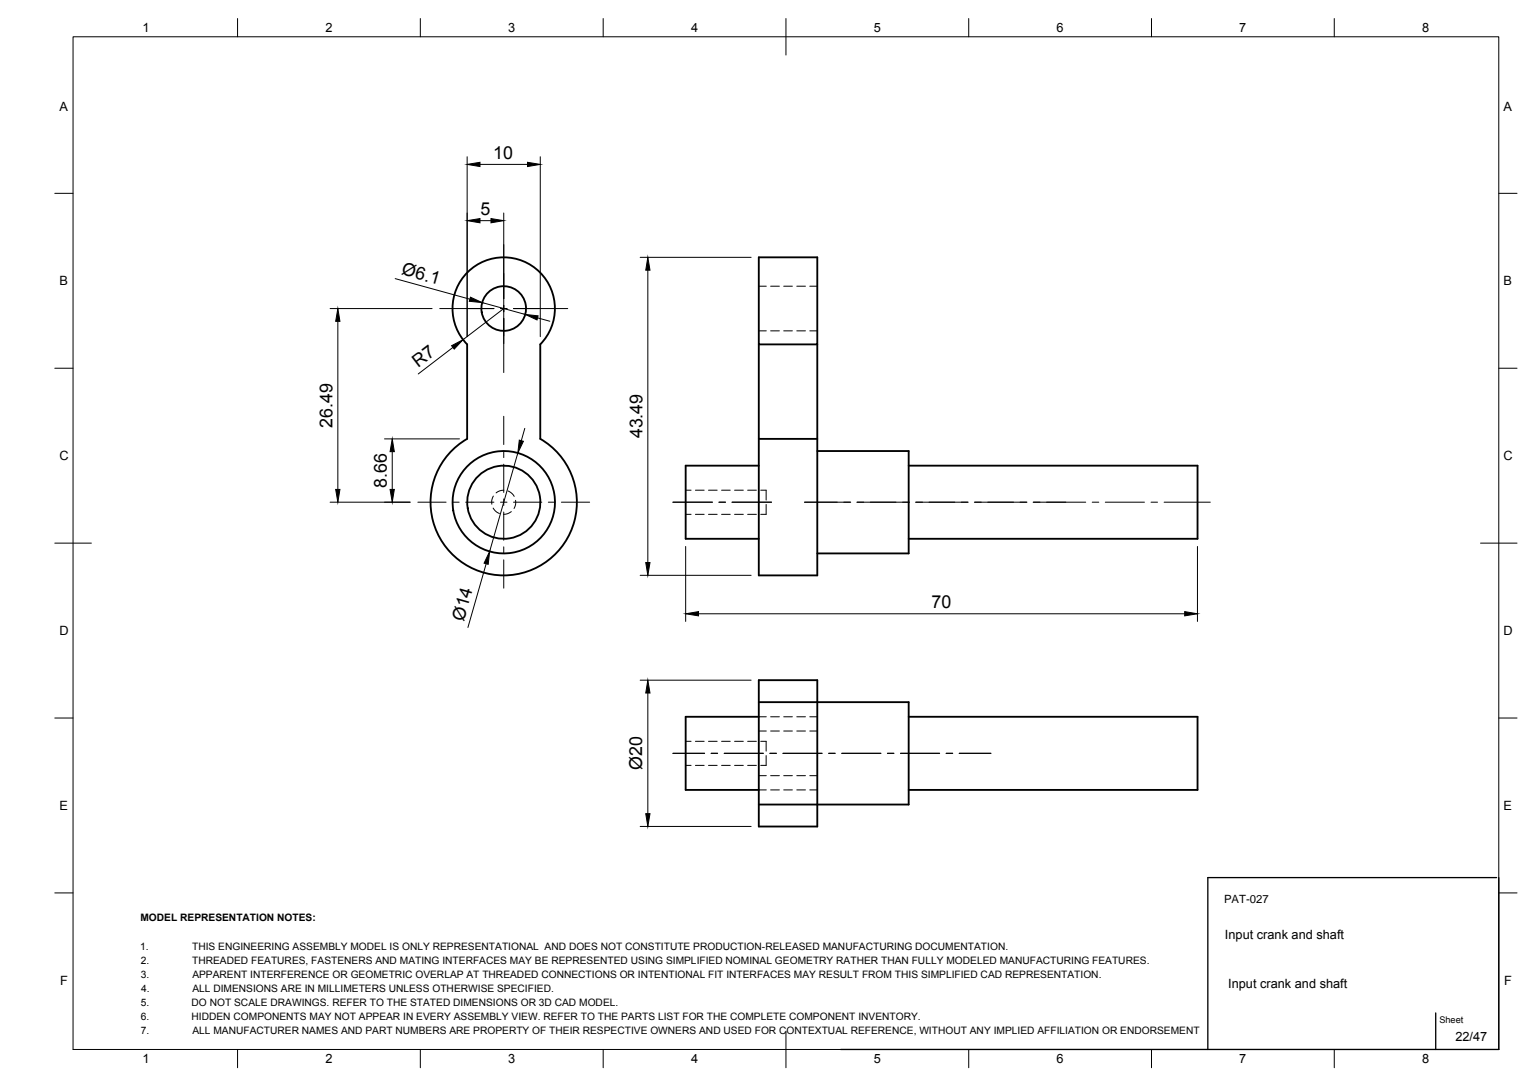
ISO-10303-21;
HEADER;
/* Generated by software containing ST-Developer
 * from STEP Tools, Inc. (www.steptools.com) 
 */

FILE_DESCRIPTION(
/* description */ ('Crank-driven oscillating fan base (mechanism only)'),

/* implementation_level */ '2;1');

FILE_NAME(
/* name */ 'Input crank and shaft.step',
/* time_stamp */ '2026-10-28T03:25:00-07:00',
/* author */ (''),
/* organization */ (''),
/* preprocessor_version */ 'ST-DEVELOPER v20.2',
/* originating_system */ 'Autodesk Translation Framework v15.17.0.0',
/* authorisation */ '');

FILE_SCHEMA (('AUTOMOTIVE_DESIGN { 1 0 10303 214 3 1 1 }'));
ENDSEC;

DATA;
#10=MECHANICAL_DESIGN_GEOMETRIC_PRESENTATION_REPRESENTATION('',(#459),#11916);
#371=SHAPE_REPRESENTATION_RELATIONSHIP('SRR','None',#12097,#411);
#411=ADVANCED_BREP_SHAPE_REPRESENTATION('',(#506),#11888);
#459=STYLED_ITEM('',(#12375),#506);
#506=MANIFOLD_SOLID_BREP('Body1',#6090);
#616=FACE_BOUND('',#1528,.T.);
#617=FACE_BOUND('',#1529,.T.);
#618=FACE_BOUND('',#1533,.T.);
#619=FACE_BOUND('',#1534,.T.);
#620=FACE_BOUND('',#1536,.T.);
#621=FACE_BOUND('',#1541,.T.);
#770=PLANE('',#6968);
#771=PLANE('',#6975);
#772=PLANE('',#6976);
#773=PLANE('',#6979);
#774=PLANE('',#6982);
#775=PLANE('',#6984);
#776=PLANE('',#6992);
#777=PLANE('',#6993);
#1061=FACE_OUTER_BOUND('',#1522,.T.);
#1062=FACE_OUTER_BOUND('',#1523,.T.);
#1063=FACE_OUTER_BOUND('',#1524,.T.);
#1064=FACE_OUTER_BOUND('',#1525,.T.);
#1065=FACE_OUTER_BOUND('',#1526,.T.);
#1066=FACE_OUTER_BOUND('',#1527,.T.);
#1067=FACE_OUTER_BOUND('',#1530,.T.);
#1068=FACE_OUTER_BOUND('',#1531,.T.);
#1069=FACE_OUTER_BOUND('',#1532,.T.);
#1070=FACE_OUTER_BOUND('',#1535,.T.);
#1071=FACE_OUTER_BOUND('',#1537,.T.);
#1072=FACE_OUTER_BOUND('',#1538,.T.);
#1073=FACE_OUTER_BOUND('',#1539,.T.);
#1074=FACE_OUTER_BOUND('',#1540,.T.);
#1075=FACE_OUTER_BOUND('',#1542,.T.);
#1522=EDGE_LOOP('',(#4816,#4817,#4818,#4819));
#1523=EDGE_LOOP('',(#4820));
#1524=EDGE_LOOP('',(#4821,#4822,#4823,#4824));
#1525=EDGE_LOOP('',(#4825,#4826,#4827,#4828));
#1526=EDGE_LOOP('',(#4829,#4830,#4831,#4832));
#1527=EDGE_LOOP('',(#4833,#4834,#4835,#4836));
#1528=EDGE_LOOP('',(#4837));
#1529=EDGE_LOOP('',(#4838));
#1530=EDGE_LOOP('',(#4839,#4840,#4841,#4842));
#1531=EDGE_LOOP('',(#4843,#4844,#4845,#4846));
#1532=EDGE_LOOP('',(#4847,#4848,#4849,#4850));
#1533=EDGE_LOOP('',(#4851));
#1534=EDGE_LOOP('',(#4852));
#1535=EDGE_LOOP('',(#4853));
#1536=EDGE_LOOP('',(#4854));
#1537=EDGE_LOOP('',(#4855,#4856,#4857,#4858));
#1538=EDGE_LOOP('',(#4859,#4860,#4861,#4862));
#1539=EDGE_LOOP('',(#4863,#4864,#4865,#4866));
#1540=EDGE_LOOP('',(#4867));
#1541=EDGE_LOOP('',(#4868));
#1542=EDGE_LOOP('',(#4869));
#1939=LINE('',#10758,#2272);
#1940=LINE('',#10765,#2273);
#1941=LINE('',#10770,#2274);
#1942=LINE('',#10774,#2275);
#1943=LINE('',#10778,#2276);
#1944=LINE('',#10780,#2277);
#1945=LINE('',#10781,#2278);
#1946=LINE('',#10784,#2279);
#1947=LINE('',#10790,#2280);
#1948=LINE('',#10791,#2281);
#1949=LINE('',#10803,#2282);
#1950=LINE('',#10806,#2283);
#1951=LINE('',#10811,#2284);
#2272=VECTOR('',#8368,0.165);
#2273=VECTOR('',#8377,0.305);
#2274=VECTOR('',#8382,1.);
#2275=VECTOR('',#8385,1.);
#2276=VECTOR('',#8390,1.);
#2277=VECTOR('',#8391,1.);
#2278=VECTOR('',#8392,1.);
#2279=VECTOR('',#8395,1.);
#2280=VECTOR('',#8402,1.);
#2281=VECTOR('',#8403,1.);
#2282=VECTOR('',#8420,0.7);
#2283=VECTOR('',#8423,0.5);
#2284=VECTOR('',#8430,0.5);
#2671=CIRCLE('',#6966,0.165);
#2672=CIRCLE('',#6967,0.165);
#2673=CIRCLE('',#6970,0.305);
#2674=CIRCLE('',#6971,0.305);
#2675=CIRCLE('',#6973,0.7);
#2676=CIRCLE('',#6974,0.7);
#2677=CIRCLE('',#6977,1.);
#2678=CIRCLE('',#6978,0.5);
#2679=CIRCLE('',#6981,1.);
#2680=CIRCLE('',#6983,0.7);
#2681=CIRCLE('',#6985,0.7);
#2682=CIRCLE('',#6986,0.5);
#2683=CIRCLE('',#6989,0.5);
#2684=CIRCLE('',#6991,0.5);
#3088=VERTEX_POINT('',#10755);
#3089=VERTEX_POINT('',#10757);
#3090=VERTEX_POINT('',#10762);
#3091=VERTEX_POINT('',#10764);
#3092=VERTEX_POINT('',#10768);
#3093=VERTEX_POINT('',#10769);
#3094=VERTEX_POINT('',#10771);
#3095=VERTEX_POINT('',#10773);
#3096=VERTEX_POINT('',#10777);
#3097=VERTEX_POINT('',#10779);
#3098=VERTEX_POINT('',#10783);
#3099=VERTEX_POINT('',#10786);
#3100=VERTEX_POINT('',#10789);
#3101=VERTEX_POINT('',#10795);
#3102=VERTEX_POINT('',#10798);
#3103=VERTEX_POINT('',#10800);
#3104=VERTEX_POINT('',#10805);
#3105=VERTEX_POINT('',#10809);
#3703=EDGE_CURVE('',#3088,#3088,#2671,.T.);
#3704=EDGE_CURVE('',#3088,#3089,#1939,.T.);
#3705=EDGE_CURVE('',#3089,#3089,#2672,.T.);
#3706=EDGE_CURVE('',#3090,#3090,#2673,.T.);
#3707=EDGE_CURVE('',#3090,#3091,#1940,.T.);
#3708=EDGE_CURVE('',#3091,#3091,#2674,.T.);
#3709=EDGE_CURVE('',#3092,#3093,#1941,.T.);
#3710=EDGE_CURVE('',#3092,#3094,#2675,.T.);
#3711=EDGE_CURVE('',#3095,#3094,#1942,.T.);
#3712=EDGE_CURVE('',#3093,#3095,#2676,.T.);
#3713=EDGE_CURVE('',#3096,#3093,#1943,.T.);
#3714=EDGE_CURVE('',#3097,#3096,#1944,.T.);
#3715=EDGE_CURVE('',#3092,#3097,#1945,.T.);
#3716=EDGE_CURVE('',#3095,#3098,#1946,.T.);
#3717=EDGE_CURVE('',#3098,#3096,#2677,.T.);
#3718=EDGE_CURVE('',#3099,#3099,#2678,.T.);
#3719=EDGE_CURVE('',#3100,#3094,#1947,.T.);
#3720=EDGE_CURVE('',#3098,#3100,#1948,.T.);
#3721=EDGE_CURVE('',#3100,#3097,#2679,.T.);
#3722=EDGE_CURVE('',#3101,#3101,#2680,.T.);
#3723=EDGE_CURVE('',#3102,#3102,#2681,.T.);
#3724=EDGE_CURVE('',#3103,#3103,#2682,.T.);
#3725=EDGE_CURVE('',#3101,#3102,#1949,.T.);
#3726=EDGE_CURVE('',#3103,#3104,#1950,.T.);
#3727=EDGE_CURVE('',#3104,#3104,#2683,.T.);
#3728=EDGE_CURVE('',#3105,#3105,#2684,.T.);
#3729=EDGE_CURVE('',#3105,#3099,#1951,.T.);
#4816=ORIENTED_EDGE('',*,*,#3703,.F.);
#4817=ORIENTED_EDGE('',*,*,#3704,.T.);
#4818=ORIENTED_EDGE('',*,*,#3705,.F.);
#4819=ORIENTED_EDGE('',*,*,#3704,.F.);
#4820=ORIENTED_EDGE('',*,*,#3703,.T.);
#4821=ORIENTED_EDGE('',*,*,#3706,.F.);
#4822=ORIENTED_EDGE('',*,*,#3707,.T.);
#4823=ORIENTED_EDGE('',*,*,#3708,.F.);
#4824=ORIENTED_EDGE('',*,*,#3707,.F.);
#4825=ORIENTED_EDGE('',*,*,#3709,.F.);
#4826=ORIENTED_EDGE('',*,*,#3710,.T.);
#4827=ORIENTED_EDGE('',*,*,#3711,.F.);
#4828=ORIENTED_EDGE('',*,*,#3712,.F.);
#4829=ORIENTED_EDGE('',*,*,#3709,.T.);
#4830=ORIENTED_EDGE('',*,*,#3713,.F.);
#4831=ORIENTED_EDGE('',*,*,#3714,.F.);
#4832=ORIENTED_EDGE('',*,*,#3715,.F.);
#4833=ORIENTED_EDGE('',*,*,#3712,.T.);
#4834=ORIENTED_EDGE('',*,*,#3716,.T.);
#4835=ORIENTED_EDGE('',*,*,#3717,.T.);
#4836=ORIENTED_EDGE('',*,*,#3713,.T.);
#4837=ORIENTED_EDGE('',*,*,#3708,.T.);
#4838=ORIENTED_EDGE('',*,*,#3718,.F.);
#4839=ORIENTED_EDGE('',*,*,#3711,.T.);
#4840=ORIENTED_EDGE('',*,*,#3719,.F.);
#4841=ORIENTED_EDGE('',*,*,#3720,.F.);
#4842=ORIENTED_EDGE('',*,*,#3716,.F.);
#4843=ORIENTED_EDGE('',*,*,#3720,.T.);
#4844=ORIENTED_EDGE('',*,*,#3721,.T.);
#4845=ORIENTED_EDGE('',*,*,#3714,.T.);
#4846=ORIENTED_EDGE('',*,*,#3717,.F.);
#4847=ORIENTED_EDGE('',*,*,#3715,.T.);
#4848=ORIENTED_EDGE('',*,*,#3721,.F.);
#4849=ORIENTED_EDGE('',*,*,#3719,.T.);
#4850=ORIENTED_EDGE('',*,*,#3710,.F.);
#4851=ORIENTED_EDGE('',*,*,#3706,.T.);
#4852=ORIENTED_EDGE('',*,*,#3722,.T.);
#4853=ORIENTED_EDGE('',*,*,#3723,.F.);
#4854=ORIENTED_EDGE('',*,*,#3724,.F.);
#4855=ORIENTED_EDGE('',*,*,#3722,.F.);
#4856=ORIENTED_EDGE('',*,*,#3725,.T.);
#4857=ORIENTED_EDGE('',*,*,#3723,.T.);
#4858=ORIENTED_EDGE('',*,*,#3725,.F.);
#4859=ORIENTED_EDGE('',*,*,#3724,.T.);
#4860=ORIENTED_EDGE('',*,*,#3726,.T.);
#4861=ORIENTED_EDGE('',*,*,#3727,.T.);
#4862=ORIENTED_EDGE('',*,*,#3726,.F.);
#4863=ORIENTED_EDGE('',*,*,#3728,.F.);
#4864=ORIENTED_EDGE('',*,*,#3729,.T.);
#4865=ORIENTED_EDGE('',*,*,#3718,.T.);
#4866=ORIENTED_EDGE('',*,*,#3729,.F.);
#4867=ORIENTED_EDGE('',*,*,#3728,.T.);
#4868=ORIENTED_EDGE('',*,*,#3705,.T.);
#4869=ORIENTED_EDGE('',*,*,#3727,.F.);
#5618=CYLINDRICAL_SURFACE('',#6965,0.165);
#5619=CYLINDRICAL_SURFACE('',#6969,0.305);
#5620=CYLINDRICAL_SURFACE('',#6972,0.7);
#5621=CYLINDRICAL_SURFACE('',#6980,1.);
#5622=CYLINDRICAL_SURFACE('',#6987,0.7);
#5623=CYLINDRICAL_SURFACE('',#6988,0.5);
#5624=CYLINDRICAL_SURFACE('',#6990,0.5);
#5867=ADVANCED_FACE('',(#1061),#5618,.F.);
#5868=ADVANCED_FACE('',(#1062),#770,.T.);
#5869=ADVANCED_FACE('',(#1063),#5619,.F.);
#5870=ADVANCED_FACE('',(#1064),#5620,.T.);
#5871=ADVANCED_FACE('',(#1065),#771,.T.);
#5872=ADVANCED_FACE('',(#1066,#616,#617),#772,.T.);
#5873=ADVANCED_FACE('',(#1067),#773,.T.);
#5874=ADVANCED_FACE('',(#1068),#5621,.T.);
#5875=ADVANCED_FACE('',(#1069,#618,#619),#774,.F.);
#5876=ADVANCED_FACE('',(#1070,#620),#775,.F.);
#5877=ADVANCED_FACE('',(#1071),#5622,.T.);
#5878=ADVANCED_FACE('',(#1072),#5623,.T.);
#5879=ADVANCED_FACE('',(#1073),#5624,.T.);
#5880=ADVANCED_FACE('',(#1074,#621),#776,.T.);
#5881=ADVANCED_FACE('',(#1075),#777,.F.);
#6090=CLOSED_SHELL('',(#5867,#5868,#5869,#5870,#5871,#5872,#5873,#5874,
#5875,#5876,#5877,#5878,#5879,#5880,#5881));
#6964=AXIS2_PLACEMENT_3D('',#10753,#8362,#8363);
#6965=AXIS2_PLACEMENT_3D('',#10754,#8364,#8365);
#6966=AXIS2_PLACEMENT_3D('',#10756,#8366,#8367);
#6967=AXIS2_PLACEMENT_3D('',#10759,#8369,#8370);
#6968=AXIS2_PLACEMENT_3D('',#10760,#8371,#8372);
#6969=AXIS2_PLACEMENT_3D('',#10761,#8373,#8374);
#6970=AXIS2_PLACEMENT_3D('',#10763,#8375,#8376);
#6971=AXIS2_PLACEMENT_3D('',#10766,#8378,#8379);
#6972=AXIS2_PLACEMENT_3D('',#10767,#8380,#8381);
#6973=AXIS2_PLACEMENT_3D('',#10772,#8383,#8384);
#6974=AXIS2_PLACEMENT_3D('',#10775,#8386,#8387);
#6975=AXIS2_PLACEMENT_3D('',#10776,#8388,#8389);
#6976=AXIS2_PLACEMENT_3D('',#10782,#8393,#8394);
#6977=AXIS2_PLACEMENT_3D('',#10785,#8396,#8397);
#6978=AXIS2_PLACEMENT_3D('',#10787,#8398,#8399);
#6979=AXIS2_PLACEMENT_3D('',#10788,#8400,#8401);
#6980=AXIS2_PLACEMENT_3D('',#10792,#8404,#8405);
#6981=AXIS2_PLACEMENT_3D('',#10793,#8406,#8407);
#6982=AXIS2_PLACEMENT_3D('',#10794,#8408,#8409);
#6983=AXIS2_PLACEMENT_3D('',#10796,#8410,#8411);
#6984=AXIS2_PLACEMENT_3D('',#10797,#8412,#8413);
#6985=AXIS2_PLACEMENT_3D('',#10799,#8414,#8415);
#6986=AXIS2_PLACEMENT_3D('',#10801,#8416,#8417);
#6987=AXIS2_PLACEMENT_3D('',#10802,#8418,#8419);
#6988=AXIS2_PLACEMENT_3D('',#10804,#8421,#8422);
#6989=AXIS2_PLACEMENT_3D('',#10807,#8424,#8425);
#6990=AXIS2_PLACEMENT_3D('',#10808,#8426,#8427);
#6991=AXIS2_PLACEMENT_3D('',#10810,#8428,#8429);
#6992=AXIS2_PLACEMENT_3D('',#10812,#8431,#8432);
#6993=AXIS2_PLACEMENT_3D('',#10813,#8433,#8434);
#8362=DIRECTION('axis',(0.,0.,1.));
#8363=DIRECTION('refdir',(1.,0.,0.));
#8364=DIRECTION('center_axis',(0.,0.,1.));
#8365=DIRECTION('ref_axis',(1.,0.,0.));
#8366=DIRECTION('center_axis',(0.,0.,1.));
#8367=DIRECTION('ref_axis',(1.,0.,0.));
#8368=DIRECTION('',(0.,0.,1.));
#8369=DIRECTION('center_axis',(0.,0.,-1.));
#8370=DIRECTION('ref_axis',(1.,0.,0.));
#8371=DIRECTION('center_axis',(0.,0.,1.));
#8372=DIRECTION('ref_axis',(1.,0.,0.));
#8373=DIRECTION('center_axis',(0.,0.,1.));
#8374=DIRECTION('ref_axis',(1.,0.,0.));
#8375=DIRECTION('center_axis',(0.,0.,1.));
#8376=DIRECTION('ref_axis',(1.,0.,0.));
#8377=DIRECTION('',(0.,0.,1.));
#8378=DIRECTION('center_axis',(0.,0.,-1.));
#8379=DIRECTION('ref_axis',(1.,0.,0.));
#8380=DIRECTION('center_axis',(0.,0.,1.));
#8381=DIRECTION('ref_axis',(-0.162294462269189,0.986742371400334,0.));
#8382=DIRECTION('',(0.,0.,1.));
#8383=DIRECTION('center_axis',(0.,0.,1.));
#8384=DIRECTION('ref_axis',(1.,0.,0.));
#8385=DIRECTION('',(0.,0.,-1.));
#8386=DIRECTION('center_axis',(0.,0.,1.));
#8387=DIRECTION('ref_axis',(1.,0.,0.));
#8388=DIRECTION('center_axis',(0.986742371400334,0.162294462269189,0.));
#8389=DIRECTION('ref_axis',(-0.162294462269189,0.986742371400334,0.));
#8390=DIRECTION('',(-0.162294462269189,0.986742371400334,0.));
#8391=DIRECTION('',(0.,0.,1.));
#8392=DIRECTION('',(0.162294462269189,-0.986742371400334,0.));
#8393=DIRECTION('center_axis',(0.,0.,1.));
#8394=DIRECTION('ref_axis',(1.,0.,0.));
#8395=DIRECTION('',(0.162294462269189,-0.986742371400334,0.));
#8396=DIRECTION('center_axis',(0.,0.,1.));
#8397=DIRECTION('ref_axis',(1.,0.,0.));
#8398=DIRECTION('center_axis',(0.,0.,1.));
#8399=DIRECTION('ref_axis',(1.,0.,0.));
#8400=DIRECTION('center_axis',(-0.986742371400334,-0.162294462269189,0.));
#8401=DIRECTION('ref_axis',(0.162294462269189,-0.986742371400334,0.));
#8402=DIRECTION('',(-0.162294462269189,0.986742371400334,0.));
#8403=DIRECTION('',(0.,0.,-1.));
#8404=DIRECTION('center_axis',(0.,0.,1.));
#8405=DIRECTION('ref_axis',(0.162294462269189,-0.986742371400334,0.));
#8406=DIRECTION('center_axis',(0.,0.,1.));
#8407=DIRECTION('ref_axis',(1.,0.,0.));
#8408=DIRECTION('center_axis',(0.,0.,1.));
#8409=DIRECTION('ref_axis',(1.,0.,0.));
#8410=DIRECTION('center_axis',(0.,0.,1.));
#8411=DIRECTION('ref_axis',(1.,0.,0.));
#8412=DIRECTION('center_axis',(0.,0.,1.));
#8413=DIRECTION('ref_axis',(1.,0.,0.));
#8414=DIRECTION('center_axis',(0.,0.,1.));
#8415=DIRECTION('ref_axis',(1.,0.,0.));
#8416=DIRECTION('center_axis',(0.,0.,-1.));
#8417=DIRECTION('ref_axis',(1.,0.,0.));
#8418=DIRECTION('center_axis',(0.,0.,1.));
#8419=DIRECTION('ref_axis',(1.,0.,0.));
#8420=DIRECTION('',(0.,0.,-1.));
#8421=DIRECTION('center_axis',(0.,0.,1.));
#8422=DIRECTION('ref_axis',(1.,0.,0.));
#8423=DIRECTION('',(0.,0.,-1.));
#8424=DIRECTION('center_axis',(0.,0.,1.));
#8425=DIRECTION('ref_axis',(1.,0.,0.));
#8426=DIRECTION('center_axis',(0.,0.,1.));
#8427=DIRECTION('ref_axis',(1.,0.,0.));
#8428=DIRECTION('center_axis',(0.,0.,1.));
#8429=DIRECTION('ref_axis',(1.,0.,0.));
#8430=DIRECTION('',(0.,0.,-1.));
#8431=DIRECTION('center_axis',(0.,0.,1.));
#8432=DIRECTION('ref_axis',(1.,0.,0.));
#8433=DIRECTION('center_axis',(0.,0.,1.));
#8434=DIRECTION('ref_axis',(1.,0.,0.));
#10753=CARTESIAN_POINT('',(0.,0.,0.));
#10754=CARTESIAN_POINT('Origin',(0.,0.,6.9));
#10755=CARTESIAN_POINT('',(-0.165,-2.02066721859313E-17,6.9));
#10756=CARTESIAN_POINT('Origin',(0.,0.,6.9));
#10757=CARTESIAN_POINT('',(-0.165,2.02066721859313E-17,8.));
#10758=CARTESIAN_POINT('',(-0.165,-2.02066721859313E-17,6.9));
#10759=CARTESIAN_POINT('Origin',(0.,0.,8.));
#10760=CARTESIAN_POINT('Origin',(0.,0.,6.9));
#10761=CARTESIAN_POINT('Origin',(-0.429855350392604,2.61349944954989,6.1));
#10762=CARTESIAN_POINT('',(-0.734855350392604,2.61349944954989,6.2));
#10763=CARTESIAN_POINT('Origin',(-0.429855350392604,2.61349944954989,6.2));
#10764=CARTESIAN_POINT('',(-0.734855350392604,2.61349944954989,7.));
#10765=CARTESIAN_POINT('',(-0.734855350392604,2.61349944954989,6.1));
#10766=CARTESIAN_POINT('Origin',(-0.429855350392604,2.61349944954989,7.));
#10767=CARTESIAN_POINT('Origin',(-0.429855350392604,2.61349944954989,6.2));
#10768=CARTESIAN_POINT('',(0.143023559435341,2.21124361718155,6.2));
#10769=CARTESIAN_POINT('',(0.143023559435341,2.21124361718155,7.));
#10770=CARTESIAN_POINT('',(0.143023559435341,2.21124361718155,6.2));
#10771=CARTESIAN_POINT('',(-0.843718811964994,2.04894915491236,6.2));
#10772=CARTESIAN_POINT('Origin',(-0.429855350392604,2.61349944954989,6.2));
#10773=CARTESIAN_POINT('',(-0.843718811964994,2.04894915491236,7.));
#10774=CARTESIAN_POINT('',(-0.843718811964994,2.04894915491236,6.2));
#10775=CARTESIAN_POINT('Origin',(-0.429855350392604,2.61349944954989,7.));
#10776=CARTESIAN_POINT('Origin',(0.493371185700167,0.0811472311345947,6.2));
#10777=CARTESIAN_POINT('',(0.352820058481515,0.935691191757783,7.));
#10778=CARTESIAN_POINT('',(0.0635158353075629,2.69464668068448,7.));
#10779=CARTESIAN_POINT('',(0.352820058481515,0.935691191757783,6.2));
#10780=CARTESIAN_POINT('',(0.352820058481515,0.935691191757783,6.2));
#10781=CARTESIAN_POINT('',(0.0635158353075629,2.69464668068448,6.2));
#10782=CARTESIAN_POINT('Origin',(0.,0.,7.));
#10783=CARTESIAN_POINT('',(-0.63392231291882,0.773396729488594,7.));
#10784=CARTESIAN_POINT('',(-0.493371185700167,-0.0811472311345944,7.));
#10785=CARTESIAN_POINT('Origin',(0.,0.,7.));
#10786=CARTESIAN_POINT('',(-0.5,-6.12323399573677E-17,7.));
#10787=CARTESIAN_POINT('Origin',(0.,0.,7.));
#10788=CARTESIAN_POINT('Origin',(-0.923226536092771,2.53235221841529,6.2));
#10789=CARTESIAN_POINT('',(-0.63392231291882,0.773396729488594,6.2));
#10790=CARTESIAN_POINT('',(-0.493371185700167,-0.0811472311345944,6.2));
#10791=CARTESIAN_POINT('',(-0.63392231291882,0.773396729488594,6.2));
#10792=CARTESIAN_POINT('Origin',(0.,0.,6.2));
#10793=CARTESIAN_POINT('Origin',(0.,0.,6.2));
#10794=CARTESIAN_POINT('Origin',(0.,0.,6.2));
#10795=CARTESIAN_POINT('',(-0.7,-8.57252759403147E-17,6.2));
#10796=CARTESIAN_POINT('Origin',(0.,0.,6.2));
#10797=CARTESIAN_POINT('Origin',(0.,0.,4.95));
#10798=CARTESIAN_POINT('',(-0.7,-8.57252759403147E-17,4.95));
#10799=CARTESIAN_POINT('Origin',(0.,0.,4.95));
#10800=CARTESIAN_POINT('',(-0.5,6.12323399573677E-17,4.95));
#10801=CARTESIAN_POINT('Origin',(0.,0.,4.95));
#10802=CARTESIAN_POINT('Origin',(0.,0.,4.95));
#10803=CARTESIAN_POINT('',(-0.7,-8.57252759403147E-17,4.95));
#10804=CARTESIAN_POINT('Origin',(0.,0.,1.));
#10805=CARTESIAN_POINT('',(-0.5,-6.12323399573677E-17,1.));
#10806=CARTESIAN_POINT('',(-0.5,-6.12323399573677E-17,1.));
#10807=CARTESIAN_POINT('Origin',(0.,0.,1.));
#10808=CARTESIAN_POINT('Origin',(0.,0.,1.));
#10809=CARTESIAN_POINT('',(-0.5,-6.12323399573677E-17,8.));
#10810=CARTESIAN_POINT('Origin',(0.,0.,8.));
#10811=CARTESIAN_POINT('',(-0.5,-6.12323399573677E-17,1.));
#10812=CARTESIAN_POINT('Origin',(0.,0.,8.));
#10813=CARTESIAN_POINT('Origin',(0.,0.,1.));
#11841=UNCERTAINTY_MEASURE_WITH_UNIT(LENGTH_MEASURE(0.001),#11917,
'DISTANCE_ACCURACY_VALUE',
'Maximum model space distance between geometric entities at asserted c
onnectivities');
#11869=UNCERTAINTY_MEASURE_WITH_UNIT(LENGTH_MEASURE(0.001),#11917,
'DISTANCE_ACCURACY_VALUE',
'Maximum model space distance between geometric entities at asserted c
onnectivities');
#11888=(
GEOMETRIC_REPRESENTATION_CONTEXT(3)
GLOBAL_UNCERTAINTY_ASSIGNED_CONTEXT((#11841))
GLOBAL_UNIT_ASSIGNED_CONTEXT((#11917,#11919,#11920))
REPRESENTATION_CONTEXT('','3D')
);
#11916=(
GEOMETRIC_REPRESENTATION_CONTEXT(3)
GLOBAL_UNCERTAINTY_ASSIGNED_CONTEXT((#11869))
GLOBAL_UNIT_ASSIGNED_CONTEXT((#11917,#11919,#11920))
REPRESENTATION_CONTEXT('','3D')
);
#11917=(
LENGTH_UNIT()
NAMED_UNIT(*)
SI_UNIT(.CENTI.,.METRE.)
);
#11919=(
NAMED_UNIT(*)
PLANE_ANGLE_UNIT()
SI_UNIT($,.RADIAN.)
);
#11920=(
NAMED_UNIT(*)
SI_UNIT($,.STERADIAN.)
SOLID_ANGLE_UNIT()
);
#11939=SHAPE_DEFINITION_REPRESENTATION(#11990,#12097);
#11990=PRODUCT_DEFINITION_SHAPE('',$,#12144);
#12097=SHAPE_REPRESENTATION('',(#6964),#11888);
#12125=PRODUCT_DEFINITION_CONTEXT('part definition',#12265,'design');
#12144=PRODUCT_DEFINITION('Input crank and shaft',
'Input crank and shaft',#12190,#12125);
#12190=PRODUCT_DEFINITION_FORMATION('',$,#12285);
#12265=APPLICATION_CONTEXT(
'Core Data for Automotive Mechanical Design Process');
#12266=PRODUCT_CONTEXT('part definition',#12265,'mechanical');
#12285=PRODUCT('Input crank and shaft','Input crank and shaft',
'Input crank and shaft',(#12266));
#12369=COLOUR_RGB('Grey',0.48,0.52,0.57);
#12370=FILL_AREA_STYLE_COLOUR('',#12369);
#12371=FILL_AREA_STYLE('',(#12370));
#12372=SURFACE_STYLE_FILL_AREA(#12371);
#12373=SURFACE_SIDE_STYLE('',(#12372));
#12374=SURFACE_STYLE_USAGE(.BOTH.,#12373);
#12375=PRESENTATION_STYLE_ASSIGNMENT((#12374));
ENDSEC;
END-ISO-10303-21;
